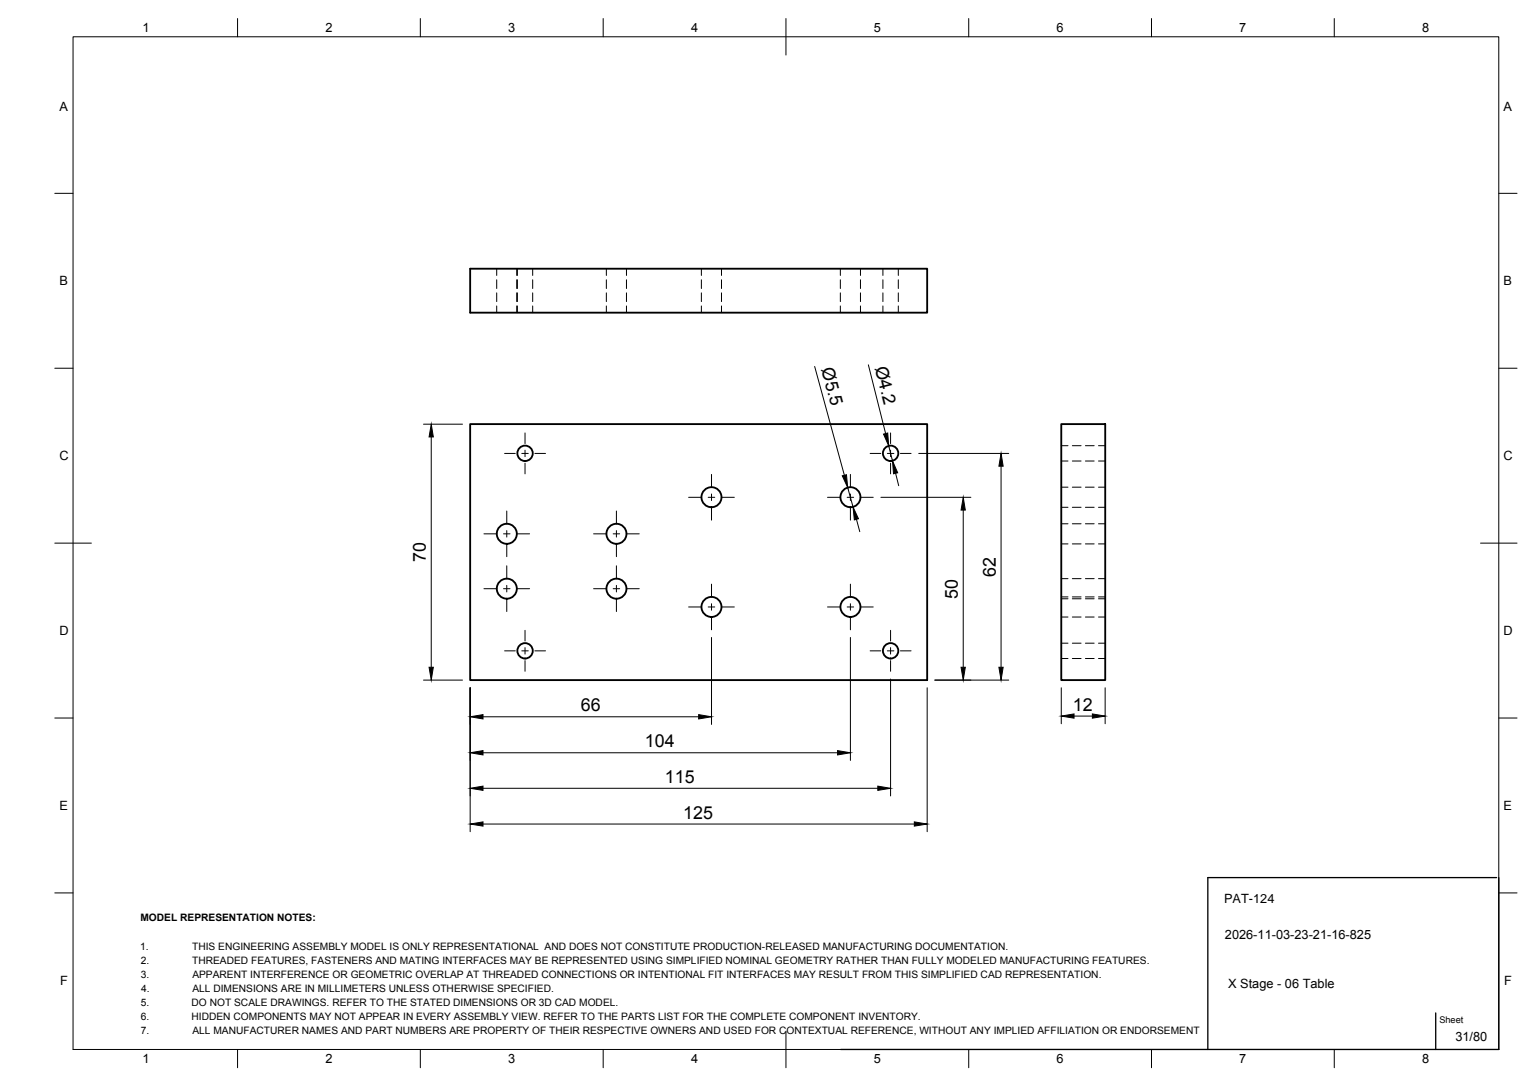
ISO-10303-21;
HEADER;
/* Generated by software containing ST-Developer
 * from STEP Tools, Inc. (www.steptools.com) 
 */

FILE_DESCRIPTION(
/* description */ ('XY cross-slide table'),
/* implementation_level */ '2;1');

FILE_NAME(
/* name */ 'X Stage - 06 Table.step',
/* time_stamp */ '2026-10-28T03:22:46-07:00',
/* author */ (''),
/* organization */ (''),
/* preprocessor_version */ 'ST-DEVELOPER v20.2',
/* originating_system */ 'Autodesk Translation Framework v15.17.0.0',
/* authorisation */ '');

FILE_SCHEMA (('AUTOMOTIVE_DESIGN { 1 0 10303 214 3 1 1 }'));
ENDSEC;

DATA;
#10=MECHANICAL_DESIGN_GEOMETRIC_PRESENTATION_REPRESENTATION('',(#1707),#62984);
#1526=SHAPE_REPRESENTATION_RELATIONSHIP('SRR','None',#63377,#1609);
#1609=ADVANCED_BREP_SHAPE_REPRESENTATION('',(#1820),#62914);
#1707=STYLED_ITEM('',(#63898),#1820);
#1820=MANIFOLD_SOLID_BREP('Body1',#23001);
#2009=FACE_BOUND('',#4578,.T.);
#2010=FACE_BOUND('',#4579,.T.);
#2011=FACE_BOUND('',#4580,.T.);
#2012=FACE_BOUND('',#4581,.T.);
#2013=FACE_BOUND('',#4582,.T.);
#2014=FACE_BOUND('',#4583,.T.);
#2015=FACE_BOUND('',#4584,.T.);
#2016=FACE_BOUND('',#4585,.T.);
#2017=FACE_BOUND('',#4586,.T.);
#2018=FACE_BOUND('',#4587,.T.);
#2019=FACE_BOUND('',#4588,.T.);
#2020=FACE_BOUND('',#4589,.T.);
#2021=FACE_BOUND('',#4591,.T.);
#2022=FACE_BOUND('',#4592,.T.);
#2023=FACE_BOUND('',#4593,.T.);
#2024=FACE_BOUND('',#4594,.T.);
#2025=FACE_BOUND('',#4595,.T.);
#2026=FACE_BOUND('',#4596,.T.);
#2027=FACE_BOUND('',#4597,.T.);
#2028=FACE_BOUND('',#4598,.T.);
#2029=FACE_BOUND('',#4599,.T.);
#2030=FACE_BOUND('',#4600,.T.);
#2031=FACE_BOUND('',#4601,.T.);
#2032=FACE_BOUND('',#4602,.T.);
#2420=PLANE('',#24604);
#2421=PLANE('',#24605);
#2422=PLANE('',#24606);
#2423=PLANE('',#24607);
#2424=PLANE('',#24608);
#2425=PLANE('',#24609);
#3125=FACE_OUTER_BOUND('',#4561,.T.);
#3126=FACE_OUTER_BOUND('',#4562,.T.);
#3127=FACE_OUTER_BOUND('',#4563,.T.);
#3128=FACE_OUTER_BOUND('',#4564,.T.);
#3129=FACE_OUTER_BOUND('',#4565,.T.);
#3130=FACE_OUTER_BOUND('',#4566,.T.);
#3131=FACE_OUTER_BOUND('',#4567,.T.);
#3132=FACE_OUTER_BOUND('',#4568,.T.);
#3133=FACE_OUTER_BOUND('',#4569,.T.);
#3134=FACE_OUTER_BOUND('',#4570,.T.);
#3135=FACE_OUTER_BOUND('',#4571,.T.);
#3136=FACE_OUTER_BOUND('',#4572,.T.);
#3137=FACE_OUTER_BOUND('',#4573,.T.);
#3138=FACE_OUTER_BOUND('',#4574,.T.);
#3139=FACE_OUTER_BOUND('',#4575,.T.);
#3140=FACE_OUTER_BOUND('',#4576,.T.);
#3141=FACE_OUTER_BOUND('',#4577,.T.);
#3142=FACE_OUTER_BOUND('',#4590,.T.);
#4561=EDGE_LOOP('',(#16012,#16013,#16014,#16015));
#4562=EDGE_LOOP('',(#16016,#16017,#16018,#16019));
#4563=EDGE_LOOP('',(#16020,#16021,#16022,#16023));
#4564=EDGE_LOOP('',(#16024,#16025,#16026,#16027));
#4565=EDGE_LOOP('',(#16028,#16029,#16030,#16031));
#4566=EDGE_LOOP('',(#16032,#16033,#16034,#16035));
#4567=EDGE_LOOP('',(#16036,#16037,#16038,#16039));
#4568=EDGE_LOOP('',(#16040,#16041,#16042,#16043));
#4569=EDGE_LOOP('',(#16044,#16045,#16046,#16047));
#4570=EDGE_LOOP('',(#16048,#16049,#16050,#16051));
#4571=EDGE_LOOP('',(#16052,#16053,#16054,#16055));
#4572=EDGE_LOOP('',(#16056,#16057,#16058,#16059));
#4573=EDGE_LOOP('',(#16060,#16061,#16062,#16063));
#4574=EDGE_LOOP('',(#16064,#16065,#16066,#16067));
#4575=EDGE_LOOP('',(#16068,#16069,#16070,#16071));
#4576=EDGE_LOOP('',(#16072,#16073,#16074,#16075));
#4577=EDGE_LOOP('',(#16076,#16077,#16078,#16079));
#4578=EDGE_LOOP('',(#16080));
#4579=EDGE_LOOP('',(#16081));
#4580=EDGE_LOOP('',(#16082));
#4581=EDGE_LOOP('',(#16083));
#4582=EDGE_LOOP('',(#16084));
#4583=EDGE_LOOP('',(#16085));
#4584=EDGE_LOOP('',(#16086));
#4585=EDGE_LOOP('',(#16087));
#4586=EDGE_LOOP('',(#16088));
#4587=EDGE_LOOP('',(#16089));
#4588=EDGE_LOOP('',(#16090));
#4589=EDGE_LOOP('',(#16091));
#4590=EDGE_LOOP('',(#16092,#16093,#16094,#16095));
#4591=EDGE_LOOP('',(#16096));
#4592=EDGE_LOOP('',(#16097));
#4593=EDGE_LOOP('',(#16098));
#4594=EDGE_LOOP('',(#16099));
#4595=EDGE_LOOP('',(#16100));
#4596=EDGE_LOOP('',(#16101));
#4597=EDGE_LOOP('',(#16102));
#4598=EDGE_LOOP('',(#16103));
#4599=EDGE_LOOP('',(#16104));
#4600=EDGE_LOOP('',(#16105));
#4601=EDGE_LOOP('',(#16106));
#4602=EDGE_LOOP('',(#16107));
#6155=LINE('',#34739,#7642);
#6156=LINE('',#34745,#7643);
#6157=LINE('',#34751,#7644);
#6158=LINE('',#34757,#7645);
#6159=LINE('',#34763,#7646);
#6160=LINE('',#34769,#7647);
#6161=LINE('',#34775,#7648);
#6162=LINE('',#34781,#7649);
#6163=LINE('',#34787,#7650);
#6164=LINE('',#34793,#7651);
#6165=LINE('',#34799,#7652);
#6166=LINE('',#34805,#7653);
#6167=LINE('',#34810,#7654);
#6168=LINE('',#34812,#7655);
#6169=LINE('',#34814,#7656);
#6170=LINE('',#34815,#7657);
#6171=LINE('',#34818,#7658);
#6172=LINE('',#34820,#7659);
#6173=LINE('',#34821,#7660);
#6174=LINE('',#34824,#7661);
#6175=LINE('',#34826,#7662);
#6176=LINE('',#34827,#7663);
#6177=LINE('',#34829,#7664);
#6178=LINE('',#34830,#7665);
#7642=VECTOR('',#27850,0.210000000000001);
#7643=VECTOR('',#27857,0.210000000000001);
#7644=VECTOR('',#27864,0.210000000000001);
#7645=VECTOR('',#27871,0.210000000000001);
#7646=VECTOR('',#27878,0.275);
#7647=VECTOR('',#27885,0.275);
#7648=VECTOR('',#27892,0.275);
#7649=VECTOR('',#27899,0.275);
#7650=VECTOR('',#27906,0.275);
#7651=VECTOR('',#27913,0.275);
#7652=VECTOR('',#27920,0.275);
#7653=VECTOR('',#27927,0.275);
#7654=VECTOR('',#27932,1.);
#7655=VECTOR('',#27933,1.);
#7656=VECTOR('',#27934,1.);
#7657=VECTOR('',#27935,1.);
#7658=VECTOR('',#27938,1.);
#7659=VECTOR('',#27939,1.);
#7660=VECTOR('',#27940,1.);
#7661=VECTOR('',#27943,1.);
#7662=VECTOR('',#27944,1.);
#7663=VECTOR('',#27945,1.);
#7664=VECTOR('',#27948,1.);
#7665=VECTOR('',#27949,1.);
#9153=CIRCLE('',#24569,0.210000000000001);
#9154=CIRCLE('',#24570,0.210000000000001);
#9155=CIRCLE('',#24572,0.210000000000001);
#9156=CIRCLE('',#24573,0.210000000000001);
#9157=CIRCLE('',#24575,0.210000000000001);
#9158=CIRCLE('',#24576,0.210000000000001);
#9159=CIRCLE('',#24578,0.210000000000001);
#9160=CIRCLE('',#24579,0.210000000000001);
#9161=CIRCLE('',#24581,0.275);
#9162=CIRCLE('',#24582,0.275);
#9163=CIRCLE('',#24584,0.275);
#9164=CIRCLE('',#24585,0.275);
#9165=CIRCLE('',#24587,0.275);
#9166=CIRCLE('',#24588,0.275);
#9167=CIRCLE('',#24590,0.275);
#9168=CIRCLE('',#24591,0.275);
#9169=CIRCLE('',#24593,0.275);
#9170=CIRCLE('',#24594,0.275);
#9171=CIRCLE('',#24596,0.275);
#9172=CIRCLE('',#24597,0.275);
#9173=CIRCLE('',#24599,0.275);
#9174=CIRCLE('',#24600,0.275);
#9175=CIRCLE('',#24602,0.275);
#9176=CIRCLE('',#24603,0.275);
#10157=VERTEX_POINT('',#34736);
#10158=VERTEX_POINT('',#34738);
#10159=VERTEX_POINT('',#34742);
#10160=VERTEX_POINT('',#34744);
#10161=VERTEX_POINT('',#34748);
#10162=VERTEX_POINT('',#34750);
#10163=VERTEX_POINT('',#34754);
#10164=VERTEX_POINT('',#34756);
#10165=VERTEX_POINT('',#34760);
#10166=VERTEX_POINT('',#34762);
#10167=VERTEX_POINT('',#34766);
#10168=VERTEX_POINT('',#34768);
#10169=VERTEX_POINT('',#34772);
#10170=VERTEX_POINT('',#34774);
#10171=VERTEX_POINT('',#34778);
#10172=VERTEX_POINT('',#34780);
#10173=VERTEX_POINT('',#34784);
#10174=VERTEX_POINT('',#34786);
#10175=VERTEX_POINT('',#34790);
#10176=VERTEX_POINT('',#34792);
#10177=VERTEX_POINT('',#34796);
#10178=VERTEX_POINT('',#34798);
#10179=VERTEX_POINT('',#34802);
#10180=VERTEX_POINT('',#34804);
#10181=VERTEX_POINT('',#34808);
#10182=VERTEX_POINT('',#34809);
#10183=VERTEX_POINT('',#34811);
#10184=VERTEX_POINT('',#34813);
#10185=VERTEX_POINT('',#34817);
#10186=VERTEX_POINT('',#34819);
#10187=VERTEX_POINT('',#34823);
#10188=VERTEX_POINT('',#34825);
#12390=EDGE_CURVE('',#10157,#10157,#9153,.T.);
#12391=EDGE_CURVE('',#10157,#10158,#6155,.T.);
#12392=EDGE_CURVE('',#10158,#10158,#9154,.T.);
#12393=EDGE_CURVE('',#10159,#10159,#9155,.T.);
#12394=EDGE_CURVE('',#10159,#10160,#6156,.T.);
#12395=EDGE_CURVE('',#10160,#10160,#9156,.T.);
#12396=EDGE_CURVE('',#10161,#10161,#9157,.T.);
#12397=EDGE_CURVE('',#10161,#10162,#6157,.T.);
#12398=EDGE_CURVE('',#10162,#10162,#9158,.T.);
#12399=EDGE_CURVE('',#10163,#10163,#9159,.T.);
#12400=EDGE_CURVE('',#10163,#10164,#6158,.T.);
#12401=EDGE_CURVE('',#10164,#10164,#9160,.T.);
#12402=EDGE_CURVE('',#10165,#10165,#9161,.T.);
#12403=EDGE_CURVE('',#10165,#10166,#6159,.T.);
#12404=EDGE_CURVE('',#10166,#10166,#9162,.T.);
#12405=EDGE_CURVE('',#10167,#10167,#9163,.T.);
#12406=EDGE_CURVE('',#10167,#10168,#6160,.T.);
#12407=EDGE_CURVE('',#10168,#10168,#9164,.T.);
#12408=EDGE_CURVE('',#10169,#10169,#9165,.T.);
#12409=EDGE_CURVE('',#10169,#10170,#6161,.T.);
#12410=EDGE_CURVE('',#10170,#10170,#9166,.T.);
#12411=EDGE_CURVE('',#10171,#10171,#9167,.T.);
#12412=EDGE_CURVE('',#10171,#10172,#6162,.T.);
#12413=EDGE_CURVE('',#10172,#10172,#9168,.T.);
#12414=EDGE_CURVE('',#10173,#10173,#9169,.T.);
#12415=EDGE_CURVE('',#10173,#10174,#6163,.T.);
#12416=EDGE_CURVE('',#10174,#10174,#9170,.T.);
#12417=EDGE_CURVE('',#10175,#10175,#9171,.T.);
#12418=EDGE_CURVE('',#10175,#10176,#6164,.T.);
#12419=EDGE_CURVE('',#10176,#10176,#9172,.T.);
#12420=EDGE_CURVE('',#10177,#10177,#9173,.T.);
#12421=EDGE_CURVE('',#10177,#10178,#6165,.T.);
#12422=EDGE_CURVE('',#10178,#10178,#9174,.T.);
#12423=EDGE_CURVE('',#10179,#10179,#9175,.T.);
#12424=EDGE_CURVE('',#10179,#10180,#6166,.T.);
#12425=EDGE_CURVE('',#10180,#10180,#9176,.T.);
#12426=EDGE_CURVE('',#10181,#10182,#6167,.T.);
#12427=EDGE_CURVE('',#10182,#10183,#6168,.T.);
#12428=EDGE_CURVE('',#10184,#10183,#6169,.T.);
#12429=EDGE_CURVE('',#10181,#10184,#6170,.T.);
#12430=EDGE_CURVE('',#10185,#10181,#6171,.T.);
#12431=EDGE_CURVE('',#10186,#10184,#6172,.T.);
#12432=EDGE_CURVE('',#10185,#10186,#6173,.T.);
#12433=EDGE_CURVE('',#10187,#10185,#6174,.T.);
#12434=EDGE_CURVE('',#10188,#10186,#6175,.T.);
#12435=EDGE_CURVE('',#10187,#10188,#6176,.T.);
#12436=EDGE_CURVE('',#10182,#10187,#6177,.T.);
#12437=EDGE_CURVE('',#10183,#10188,#6178,.T.);
#16012=ORIENTED_EDGE('',*,*,#12390,.F.);
#16013=ORIENTED_EDGE('',*,*,#12391,.T.);
#16014=ORIENTED_EDGE('',*,*,#12392,.F.);
#16015=ORIENTED_EDGE('',*,*,#12391,.F.);
#16016=ORIENTED_EDGE('',*,*,#12393,.F.);
#16017=ORIENTED_EDGE('',*,*,#12394,.T.);
#16018=ORIENTED_EDGE('',*,*,#12395,.F.);
#16019=ORIENTED_EDGE('',*,*,#12394,.F.);
#16020=ORIENTED_EDGE('',*,*,#12396,.F.);
#16021=ORIENTED_EDGE('',*,*,#12397,.T.);
#16022=ORIENTED_EDGE('',*,*,#12398,.F.);
#16023=ORIENTED_EDGE('',*,*,#12397,.F.);
#16024=ORIENTED_EDGE('',*,*,#12399,.F.);
#16025=ORIENTED_EDGE('',*,*,#12400,.T.);
#16026=ORIENTED_EDGE('',*,*,#12401,.F.);
#16027=ORIENTED_EDGE('',*,*,#12400,.F.);
#16028=ORIENTED_EDGE('',*,*,#12402,.F.);
#16029=ORIENTED_EDGE('',*,*,#12403,.T.);
#16030=ORIENTED_EDGE('',*,*,#12404,.F.);
#16031=ORIENTED_EDGE('',*,*,#12403,.F.);
#16032=ORIENTED_EDGE('',*,*,#12405,.F.);
#16033=ORIENTED_EDGE('',*,*,#12406,.T.);
#16034=ORIENTED_EDGE('',*,*,#12407,.F.);
#16035=ORIENTED_EDGE('',*,*,#12406,.F.);
#16036=ORIENTED_EDGE('',*,*,#12408,.F.);
#16037=ORIENTED_EDGE('',*,*,#12409,.T.);
#16038=ORIENTED_EDGE('',*,*,#12410,.F.);
#16039=ORIENTED_EDGE('',*,*,#12409,.F.);
#16040=ORIENTED_EDGE('',*,*,#12411,.F.);
#16041=ORIENTED_EDGE('',*,*,#12412,.T.);
#16042=ORIENTED_EDGE('',*,*,#12413,.F.);
#16043=ORIENTED_EDGE('',*,*,#12412,.F.);
#16044=ORIENTED_EDGE('',*,*,#12414,.F.);
#16045=ORIENTED_EDGE('',*,*,#12415,.T.);
#16046=ORIENTED_EDGE('',*,*,#12416,.F.);
#16047=ORIENTED_EDGE('',*,*,#12415,.F.);
#16048=ORIENTED_EDGE('',*,*,#12417,.F.);
#16049=ORIENTED_EDGE('',*,*,#12418,.T.);
#16050=ORIENTED_EDGE('',*,*,#12419,.F.);
#16051=ORIENTED_EDGE('',*,*,#12418,.F.);
#16052=ORIENTED_EDGE('',*,*,#12420,.F.);
#16053=ORIENTED_EDGE('',*,*,#12421,.T.);
#16054=ORIENTED_EDGE('',*,*,#12422,.F.);
#16055=ORIENTED_EDGE('',*,*,#12421,.F.);
#16056=ORIENTED_EDGE('',*,*,#12423,.F.);
#16057=ORIENTED_EDGE('',*,*,#12424,.T.);
#16058=ORIENTED_EDGE('',*,*,#12425,.F.);
#16059=ORIENTED_EDGE('',*,*,#12424,.F.);
#16060=ORIENTED_EDGE('',*,*,#12426,.T.);
#16061=ORIENTED_EDGE('',*,*,#12427,.T.);
#16062=ORIENTED_EDGE('',*,*,#12428,.F.);
#16063=ORIENTED_EDGE('',*,*,#12429,.F.);
#16064=ORIENTED_EDGE('',*,*,#12430,.T.);
#16065=ORIENTED_EDGE('',*,*,#12429,.T.);
#16066=ORIENTED_EDGE('',*,*,#12431,.F.);
#16067=ORIENTED_EDGE('',*,*,#12432,.F.);
#16068=ORIENTED_EDGE('',*,*,#12433,.T.);
#16069=ORIENTED_EDGE('',*,*,#12432,.T.);
#16070=ORIENTED_EDGE('',*,*,#12434,.F.);
#16071=ORIENTED_EDGE('',*,*,#12435,.F.);
#16072=ORIENTED_EDGE('',*,*,#12436,.T.);
#16073=ORIENTED_EDGE('',*,*,#12435,.T.);
#16074=ORIENTED_EDGE('',*,*,#12437,.F.);
#16075=ORIENTED_EDGE('',*,*,#12427,.F.);
#16076=ORIENTED_EDGE('',*,*,#12437,.T.);
#16077=ORIENTED_EDGE('',*,*,#12434,.T.);
#16078=ORIENTED_EDGE('',*,*,#12431,.T.);
#16079=ORIENTED_EDGE('',*,*,#12428,.T.);
#16080=ORIENTED_EDGE('',*,*,#12404,.T.);
#16081=ORIENTED_EDGE('',*,*,#12407,.T.);
#16082=ORIENTED_EDGE('',*,*,#12410,.T.);
#16083=ORIENTED_EDGE('',*,*,#12413,.T.);
#16084=ORIENTED_EDGE('',*,*,#12416,.T.);
#16085=ORIENTED_EDGE('',*,*,#12419,.T.);
#16086=ORIENTED_EDGE('',*,*,#12422,.T.);
#16087=ORIENTED_EDGE('',*,*,#12425,.T.);
#16088=ORIENTED_EDGE('',*,*,#12401,.T.);
#16089=ORIENTED_EDGE('',*,*,#12398,.T.);
#16090=ORIENTED_EDGE('',*,*,#12395,.T.);
#16091=ORIENTED_EDGE('',*,*,#12392,.T.);
#16092=ORIENTED_EDGE('',*,*,#12436,.F.);
#16093=ORIENTED_EDGE('',*,*,#12426,.F.);
#16094=ORIENTED_EDGE('',*,*,#12430,.F.);
#16095=ORIENTED_EDGE('',*,*,#12433,.F.);
#16096=ORIENTED_EDGE('',*,*,#12402,.T.);
#16097=ORIENTED_EDGE('',*,*,#12405,.T.);
#16098=ORIENTED_EDGE('',*,*,#12408,.T.);
#16099=ORIENTED_EDGE('',*,*,#12411,.T.);
#16100=ORIENTED_EDGE('',*,*,#12414,.T.);
#16101=ORIENTED_EDGE('',*,*,#12417,.T.);
#16102=ORIENTED_EDGE('',*,*,#12420,.T.);
#16103=ORIENTED_EDGE('',*,*,#12423,.T.);
#16104=ORIENTED_EDGE('',*,*,#12399,.T.);
#16105=ORIENTED_EDGE('',*,*,#12396,.T.);
#16106=ORIENTED_EDGE('',*,*,#12393,.T.);
#16107=ORIENTED_EDGE('',*,*,#12390,.T.);
#21130=CYLINDRICAL_SURFACE('',#24568,0.210000000000001);
#21131=CYLINDRICAL_SURFACE('',#24571,0.210000000000001);
#21132=CYLINDRICAL_SURFACE('',#24574,0.210000000000001);
#21133=CYLINDRICAL_SURFACE('',#24577,0.210000000000001);
#21134=CYLINDRICAL_SURFACE('',#24580,0.275);
#21135=CYLINDRICAL_SURFACE('',#24583,0.275);
#21136=CYLINDRICAL_SURFACE('',#24586,0.275);
#21137=CYLINDRICAL_SURFACE('',#24589,0.275);
#21138=CYLINDRICAL_SURFACE('',#24592,0.275);
#21139=CYLINDRICAL_SURFACE('',#24595,0.275);
#21140=CYLINDRICAL_SURFACE('',#24598,0.275);
#21141=CYLINDRICAL_SURFACE('',#24601,0.275);
#21906=ADVANCED_FACE('',(#3125),#21130,.F.);
#21907=ADVANCED_FACE('',(#3126),#21131,.F.);
#21908=ADVANCED_FACE('',(#3127),#21132,.F.);
#21909=ADVANCED_FACE('',(#3128),#21133,.F.);
#21910=ADVANCED_FACE('',(#3129),#21134,.F.);
#21911=ADVANCED_FACE('',(#3130),#21135,.F.);
#21912=ADVANCED_FACE('',(#3131),#21136,.F.);
#21913=ADVANCED_FACE('',(#3132),#21137,.F.);
#21914=ADVANCED_FACE('',(#3133),#21138,.F.);
#21915=ADVANCED_FACE('',(#3134),#21139,.F.);
#21916=ADVANCED_FACE('',(#3135),#21140,.F.);
#21917=ADVANCED_FACE('',(#3136),#21141,.F.);
#21918=ADVANCED_FACE('',(#3137),#2420,.T.);
#21919=ADVANCED_FACE('',(#3138),#2421,.T.);
#21920=ADVANCED_FACE('',(#3139),#2422,.T.);
#21921=ADVANCED_FACE('',(#3140),#2423,.T.);
#21922=ADVANCED_FACE('',(#3141,#2009,#2010,#2011,#2012,#2013,#2014,#2015,
#2016,#2017,#2018,#2019,#2020),#2424,.T.);
#21923=ADVANCED_FACE('',(#3142,#2021,#2022,#2023,#2024,#2025,#2026,#2027,
#2028,#2029,#2030,#2031,#2032),#2425,.F.);
#23001=CLOSED_SHELL('',(#21906,#21907,#21908,#21909,#21910,#21911,#21912,
#21913,#21914,#21915,#21916,#21917,#21918,#21919,#21920,#21921,#21922,#21923));
#24567=AXIS2_PLACEMENT_3D('',#34734,#27844,#27845);
#24568=AXIS2_PLACEMENT_3D('',#34735,#27846,#27847);
#24569=AXIS2_PLACEMENT_3D('',#34737,#27848,#27849);
#24570=AXIS2_PLACEMENT_3D('',#34740,#27851,#27852);
#24571=AXIS2_PLACEMENT_3D('',#34741,#27853,#27854);
#24572=AXIS2_PLACEMENT_3D('',#34743,#27855,#27856);
#24573=AXIS2_PLACEMENT_3D('',#34746,#27858,#27859);
#24574=AXIS2_PLACEMENT_3D('',#34747,#27860,#27861);
#24575=AXIS2_PLACEMENT_3D('',#34749,#27862,#27863);
#24576=AXIS2_PLACEMENT_3D('',#34752,#27865,#27866);
#24577=AXIS2_PLACEMENT_3D('',#34753,#27867,#27868);
#24578=AXIS2_PLACEMENT_3D('',#34755,#27869,#27870);
#24579=AXIS2_PLACEMENT_3D('',#34758,#27872,#27873);
#24580=AXIS2_PLACEMENT_3D('',#34759,#27874,#27875);
#24581=AXIS2_PLACEMENT_3D('',#34761,#27876,#27877);
#24582=AXIS2_PLACEMENT_3D('',#34764,#27879,#27880);
#24583=AXIS2_PLACEMENT_3D('',#34765,#27881,#27882);
#24584=AXIS2_PLACEMENT_3D('',#34767,#27883,#27884);
#24585=AXIS2_PLACEMENT_3D('',#34770,#27886,#27887);
#24586=AXIS2_PLACEMENT_3D('',#34771,#27888,#27889);
#24587=AXIS2_PLACEMENT_3D('',#34773,#27890,#27891);
#24588=AXIS2_PLACEMENT_3D('',#34776,#27893,#27894);
#24589=AXIS2_PLACEMENT_3D('',#34777,#27895,#27896);
#24590=AXIS2_PLACEMENT_3D('',#34779,#27897,#27898);
#24591=AXIS2_PLACEMENT_3D('',#34782,#27900,#27901);
#24592=AXIS2_PLACEMENT_3D('',#34783,#27902,#27903);
#24593=AXIS2_PLACEMENT_3D('',#34785,#27904,#27905);
#24594=AXIS2_PLACEMENT_3D('',#34788,#27907,#27908);
#24595=AXIS2_PLACEMENT_3D('',#34789,#27909,#27910);
#24596=AXIS2_PLACEMENT_3D('',#34791,#27911,#27912);
#24597=AXIS2_PLACEMENT_3D('',#34794,#27914,#27915);
#24598=AXIS2_PLACEMENT_3D('',#34795,#27916,#27917);
#24599=AXIS2_PLACEMENT_3D('',#34797,#27918,#27919);
#24600=AXIS2_PLACEMENT_3D('',#34800,#27921,#27922);
#24601=AXIS2_PLACEMENT_3D('',#34801,#27923,#27924);
#24602=AXIS2_PLACEMENT_3D('',#34803,#27925,#27926);
#24603=AXIS2_PLACEMENT_3D('',#34806,#27928,#27929);
#24604=AXIS2_PLACEMENT_3D('',#34807,#27930,#27931);
#24605=AXIS2_PLACEMENT_3D('',#34816,#27936,#27937);
#24606=AXIS2_PLACEMENT_3D('',#34822,#27941,#27942);
#24607=AXIS2_PLACEMENT_3D('',#34828,#27946,#27947);
#24608=AXIS2_PLACEMENT_3D('',#34831,#27950,#27951);
#24609=AXIS2_PLACEMENT_3D('',#34832,#27952,#27953);
#27844=DIRECTION('axis',(0.,0.,1.));
#27845=DIRECTION('refdir',(1.,0.,0.));
#27846=DIRECTION('center_axis',(0.,0.,1.));
#27847=DIRECTION('ref_axis',(1.,0.,0.));
#27848=DIRECTION('center_axis',(0.,0.,1.));
#27849=DIRECTION('ref_axis',(1.,0.,0.));
#27850=DIRECTION('',(0.,0.,1.));
#27851=DIRECTION('center_axis',(0.,0.,-1.));
#27852=DIRECTION('ref_axis',(1.,0.,0.));
#27853=DIRECTION('center_axis',(0.,0.,1.));
#27854=DIRECTION('ref_axis',(1.,0.,0.));
#27855=DIRECTION('center_axis',(0.,0.,1.));
#27856=DIRECTION('ref_axis',(1.,0.,0.));
#27857=DIRECTION('',(0.,0.,1.));
#27858=DIRECTION('center_axis',(0.,0.,-1.));
#27859=DIRECTION('ref_axis',(1.,0.,0.));
#27860=DIRECTION('center_axis',(0.,0.,1.));
#27861=DIRECTION('ref_axis',(1.,0.,0.));
#27862=DIRECTION('center_axis',(0.,0.,1.));
#27863=DIRECTION('ref_axis',(1.,0.,0.));
#27864=DIRECTION('',(0.,0.,1.));
#27865=DIRECTION('center_axis',(0.,0.,-1.));
#27866=DIRECTION('ref_axis',(1.,0.,0.));
#27867=DIRECTION('center_axis',(0.,0.,1.));
#27868=DIRECTION('ref_axis',(1.,0.,0.));
#27869=DIRECTION('center_axis',(0.,0.,1.));
#27870=DIRECTION('ref_axis',(1.,0.,0.));
#27871=DIRECTION('',(0.,0.,1.));
#27872=DIRECTION('center_axis',(0.,0.,-1.));
#27873=DIRECTION('ref_axis',(1.,0.,0.));
#27874=DIRECTION('center_axis',(0.,0.,1.));
#27875=DIRECTION('ref_axis',(1.,0.,0.));
#27876=DIRECTION('center_axis',(0.,0.,1.));
#27877=DIRECTION('ref_axis',(1.,0.,0.));
#27878=DIRECTION('',(0.,0.,1.));
#27879=DIRECTION('center_axis',(0.,0.,-1.));
#27880=DIRECTION('ref_axis',(1.,0.,0.));
#27881=DIRECTION('center_axis',(0.,0.,1.));
#27882=DIRECTION('ref_axis',(1.,0.,0.));
#27883=DIRECTION('center_axis',(0.,0.,1.));
#27884=DIRECTION('ref_axis',(1.,0.,0.));
#27885=DIRECTION('',(0.,0.,1.));
#27886=DIRECTION('center_axis',(0.,0.,-1.));
#27887=DIRECTION('ref_axis',(1.,0.,0.));
#27888=DIRECTION('center_axis',(0.,0.,1.));
#27889=DIRECTION('ref_axis',(1.,0.,0.));
#27890=DIRECTION('center_axis',(0.,0.,1.));
#27891=DIRECTION('ref_axis',(1.,0.,0.));
#27892=DIRECTION('',(0.,0.,1.));
#27893=DIRECTION('center_axis',(0.,0.,-1.));
#27894=DIRECTION('ref_axis',(1.,0.,0.));
#27895=DIRECTION('center_axis',(0.,0.,1.));
#27896=DIRECTION('ref_axis',(1.,0.,0.));
#27897=DIRECTION('center_axis',(0.,0.,1.));
#27898=DIRECTION('ref_axis',(1.,0.,0.));
#27899=DIRECTION('',(0.,0.,1.));
#27900=DIRECTION('center_axis',(0.,0.,-1.));
#27901=DIRECTION('ref_axis',(1.,0.,0.));
#27902=DIRECTION('center_axis',(0.,0.,1.));
#27903=DIRECTION('ref_axis',(1.,0.,0.));
#27904=DIRECTION('center_axis',(0.,0.,1.));
#27905=DIRECTION('ref_axis',(1.,0.,0.));
#27906=DIRECTION('',(0.,0.,1.));
#27907=DIRECTION('center_axis',(0.,0.,-1.));
#27908=DIRECTION('ref_axis',(1.,0.,0.));
#27909=DIRECTION('center_axis',(0.,0.,1.));
#27910=DIRECTION('ref_axis',(1.,0.,0.));
#27911=DIRECTION('center_axis',(0.,0.,1.));
#27912=DIRECTION('ref_axis',(1.,0.,0.));
#27913=DIRECTION('',(0.,0.,1.));
#27914=DIRECTION('center_axis',(0.,0.,-1.));
#27915=DIRECTION('ref_axis',(1.,0.,0.));
#27916=DIRECTION('center_axis',(0.,0.,1.));
#27917=DIRECTION('ref_axis',(1.,0.,0.));
#27918=DIRECTION('center_axis',(0.,0.,1.));
#27919=DIRECTION('ref_axis',(1.,0.,0.));
#27920=DIRECTION('',(0.,0.,1.));
#27921=DIRECTION('center_axis',(0.,0.,-1.));
#27922=DIRECTION('ref_axis',(1.,0.,0.));
#27923=DIRECTION('center_axis',(0.,0.,1.));
#27924=DIRECTION('ref_axis',(1.,0.,0.));
#27925=DIRECTION('center_axis',(0.,0.,1.));
#27926=DIRECTION('ref_axis',(1.,0.,0.));
#27927=DIRECTION('',(0.,0.,1.));
#27928=DIRECTION('center_axis',(0.,0.,-1.));
#27929=DIRECTION('ref_axis',(1.,0.,0.));
#27930=DIRECTION('center_axis',(0.,1.,0.));
#27931=DIRECTION('ref_axis',(-1.,0.,0.));
#27932=DIRECTION('',(-1.,0.,0.));
#27933=DIRECTION('',(0.,0.,1.));
#27934=DIRECTION('',(-1.,0.,0.));
#27935=DIRECTION('',(0.,0.,1.));
#27936=DIRECTION('center_axis',(1.,0.,0.));
#27937=DIRECTION('ref_axis',(0.,1.,0.));
#27938=DIRECTION('',(0.,1.,0.));
#27939=DIRECTION('',(0.,1.,0.));
#27940=DIRECTION('',(0.,0.,1.));
#27941=DIRECTION('center_axis',(0.,-1.,0.));
#27942=DIRECTION('ref_axis',(1.,0.,0.));
#27943=DIRECTION('',(1.,0.,0.));
#27944=DIRECTION('',(1.,0.,0.));
#27945=DIRECTION('',(0.,0.,1.));
#27946=DIRECTION('center_axis',(-1.,0.,0.));
#27947=DIRECTION('ref_axis',(0.,-1.,0.));
#27948=DIRECTION('',(0.,-1.,0.));
#27949=DIRECTION('',(0.,-1.,0.));
#27950=DIRECTION('center_axis',(0.,0.,1.));
#27951=DIRECTION('ref_axis',(1.,0.,0.));
#27952=DIRECTION('center_axis',(0.,0.,1.));
#27953=DIRECTION('ref_axis',(1.,0.,0.));
#34734=CARTESIAN_POINT('',(0.,0.,0.));
#34735=CARTESIAN_POINT('Origin',(16.2,-9.,5.9));
#34736=CARTESIAN_POINT('',(15.99,-9.,6.));
#34737=CARTESIAN_POINT('Origin',(16.2,-9.,6.));
#34738=CARTESIAN_POINT('',(15.99,-9.,7.2));
#34739=CARTESIAN_POINT('',(15.99,-9.,5.9));
#34740=CARTESIAN_POINT('Origin',(16.2,-9.,7.2));
#34741=CARTESIAN_POINT('Origin',(10.8,1.,5.9));
#34742=CARTESIAN_POINT('',(10.59,1.,6.));
#34743=CARTESIAN_POINT('Origin',(10.8,1.,6.));
#34744=CARTESIAN_POINT('',(10.59,1.,7.2));
#34745=CARTESIAN_POINT('',(10.59,1.,5.9));
#34746=CARTESIAN_POINT('Origin',(10.8,1.,7.2));
#34747=CARTESIAN_POINT('Origin',(10.8,-9.,5.9));
#34748=CARTESIAN_POINT('',(10.59,-9.,6.));
#34749=CARTESIAN_POINT('Origin',(10.8,-9.,6.));
#34750=CARTESIAN_POINT('',(10.59,-9.,7.2));
#34751=CARTESIAN_POINT('',(10.59,-9.,5.9));
#34752=CARTESIAN_POINT('Origin',(10.8,-9.,7.2));
#34753=CARTESIAN_POINT('Origin',(16.2,1.,5.9));
#34754=CARTESIAN_POINT('',(15.99,1.,6.));
#34755=CARTESIAN_POINT('Origin',(16.2,1.,6.));
#34756=CARTESIAN_POINT('',(15.99,1.,7.2));
#34757=CARTESIAN_POINT('',(15.99,1.,5.9));
#34758=CARTESIAN_POINT('Origin',(16.2,1.,7.2));
#34759=CARTESIAN_POINT('Origin',(14.,-1.5,5.9));
#34760=CARTESIAN_POINT('',(13.725,-1.5,6.));
#34761=CARTESIAN_POINT('Origin',(14.,-1.5,6.));
#34762=CARTESIAN_POINT('',(13.725,-1.5,7.2));
#34763=CARTESIAN_POINT('',(13.725,-1.5,5.9));
#34764=CARTESIAN_POINT('Origin',(14.,-1.5,7.2));
#34765=CARTESIAN_POINT('Origin',(12.5,1.5,5.9));
#34766=CARTESIAN_POINT('',(12.225,1.5,6.));
#34767=CARTESIAN_POINT('Origin',(12.5,1.5,6.));
#34768=CARTESIAN_POINT('',(12.225,1.5,7.2));
#34769=CARTESIAN_POINT('',(12.225,1.5,5.9));
#34770=CARTESIAN_POINT('Origin',(12.5,1.5,7.2));
#34771=CARTESIAN_POINT('Origin',(12.5,-1.5,5.9));
#34772=CARTESIAN_POINT('',(12.225,-1.5,6.));
#34773=CARTESIAN_POINT('Origin',(12.5,-1.5,6.));
#34774=CARTESIAN_POINT('',(12.225,-1.5,7.2));
#34775=CARTESIAN_POINT('',(12.225,-1.5,5.9));
#34776=CARTESIAN_POINT('Origin',(12.5,-1.5,7.2));
#34777=CARTESIAN_POINT('Origin',(14.,1.5,5.9));
#34778=CARTESIAN_POINT('',(13.725,1.5,6.));
#34779=CARTESIAN_POINT('Origin',(14.,1.5,6.));
#34780=CARTESIAN_POINT('',(13.725,1.5,7.2));
#34781=CARTESIAN_POINT('',(13.725,1.5,5.9));
#34782=CARTESIAN_POINT('Origin',(14.,1.5,7.2));
#34783=CARTESIAN_POINT('Origin',(15.,-7.9,5.1));
#34784=CARTESIAN_POINT('',(14.725,-7.9,6.));
#34785=CARTESIAN_POINT('Origin',(15.,-7.9,6.));
#34786=CARTESIAN_POINT('',(14.725,-7.9,7.2));
#34787=CARTESIAN_POINT('',(14.725,-7.9,5.1));
#34788=CARTESIAN_POINT('Origin',(15.,-7.9,7.2));
#34789=CARTESIAN_POINT('Origin',(12.,-4.1,5.1));
#34790=CARTESIAN_POINT('',(11.725,-4.1,6.));
#34791=CARTESIAN_POINT('Origin',(12.,-4.1,6.));
#34792=CARTESIAN_POINT('',(11.725,-4.1,7.2));
#34793=CARTESIAN_POINT('',(11.725,-4.1,5.1));
#34794=CARTESIAN_POINT('Origin',(12.,-4.1,7.2));
#34795=CARTESIAN_POINT('Origin',(12.,-7.9,5.1));
#34796=CARTESIAN_POINT('',(11.725,-7.9,6.));
#34797=CARTESIAN_POINT('Origin',(12.,-7.9,6.));
#34798=CARTESIAN_POINT('',(11.725,-7.9,7.2));
#34799=CARTESIAN_POINT('',(11.725,-7.9,5.1));
#34800=CARTESIAN_POINT('Origin',(12.,-7.9,7.2));
#34801=CARTESIAN_POINT('Origin',(15.,-4.1,5.1));
#34802=CARTESIAN_POINT('',(14.725,-4.1,6.));
#34803=CARTESIAN_POINT('Origin',(15.,-4.1,6.));
#34804=CARTESIAN_POINT('',(14.725,-4.1,7.2));
#34805=CARTESIAN_POINT('',(14.725,-4.1,5.1));
#34806=CARTESIAN_POINT('Origin',(15.,-4.1,7.2));
#34807=CARTESIAN_POINT('Origin',(17.,2.5,6.));
#34808=CARTESIAN_POINT('',(17.,2.5,6.));
#34809=CARTESIAN_POINT('',(10.,2.5,6.));
#34810=CARTESIAN_POINT('',(17.,2.5,6.));
#34811=CARTESIAN_POINT('',(10.,2.5,7.2));
#34812=CARTESIAN_POINT('',(10.,2.5,6.));
#34813=CARTESIAN_POINT('',(17.,2.5,7.2));
#34814=CARTESIAN_POINT('',(17.,2.5,7.2));
#34815=CARTESIAN_POINT('',(17.,2.5,6.));
#34816=CARTESIAN_POINT('Origin',(17.,-10.,6.));
#34817=CARTESIAN_POINT('',(17.,-10.,6.));
#34818=CARTESIAN_POINT('',(17.,-10.,6.));
#34819=CARTESIAN_POINT('',(17.,-10.,7.2));
#34820=CARTESIAN_POINT('',(17.,-10.,7.2));
#34821=CARTESIAN_POINT('',(17.,-10.,6.));
#34822=CARTESIAN_POINT('Origin',(10.,-10.,6.));
#34823=CARTESIAN_POINT('',(10.,-10.,6.));
#34824=CARTESIAN_POINT('',(10.,-10.,6.));
#34825=CARTESIAN_POINT('',(10.,-10.,7.2));
#34826=CARTESIAN_POINT('',(10.,-10.,7.2));
#34827=CARTESIAN_POINT('',(10.,-10.,6.));
#34828=CARTESIAN_POINT('Origin',(10.,2.5,6.));
#34829=CARTESIAN_POINT('',(10.,2.5,6.));
#34830=CARTESIAN_POINT('',(10.,2.5,7.2));
#34831=CARTESIAN_POINT('Origin',(13.5,-3.75,7.2));
#34832=CARTESIAN_POINT('Origin',(13.5,-3.75,6.));
#62815=UNCERTAINTY_MEASURE_WITH_UNIT(LENGTH_MEASURE(0.001),#62985,
'DISTANCE_ACCURACY_VALUE',
'Maximum model space distance between geometric entities at asserted c
onnectivities');
#62885=UNCERTAINTY_MEASURE_WITH_UNIT(LENGTH_MEASURE(0.001),#62985,
'DISTANCE_ACCURACY_VALUE',
'Maximum model space distance between geometric entities at asserted c
onnectivities');
#62914=(
GEOMETRIC_REPRESENTATION_CONTEXT(3)
GLOBAL_UNCERTAINTY_ASSIGNED_CONTEXT((#62815))
GLOBAL_UNIT_ASSIGNED_CONTEXT((#62985,#62987,#62988))
REPRESENTATION_CONTEXT('','3D')
);
#62984=(
GEOMETRIC_REPRESENTATION_CONTEXT(3)
GLOBAL_UNCERTAINTY_ASSIGNED_CONTEXT((#62885))
GLOBAL_UNIT_ASSIGNED_CONTEXT((#62985,#62987,#62988))
REPRESENTATION_CONTEXT('','3D')
);
#62985=(
LENGTH_UNIT()
NAMED_UNIT(*)
SI_UNIT(.CENTI.,.METRE.)
);
#62987=(
NAMED_UNIT(*)
PLANE_ANGLE_UNIT()
SI_UNIT($,.RADIAN.)
);
#62988=(
NAMED_UNIT(*)
SI_UNIT($,.STERADIAN.)
SOLID_ANGLE_UNIT()
);
#63017=SHAPE_DEFINITION_REPRESENTATION(#63125,#63377);
#63125=PRODUCT_DEFINITION_SHAPE('',$,#63476);
#63377=SHAPE_REPRESENTATION('',(#24567),#62914);
#63447=PRODUCT_DEFINITION_CONTEXT('part definition',#63743,'design');
#63476=PRODUCT_DEFINITION('X Stage - 06 Table','X Stage - 06 Table',#63574,
#63447);
#63574=PRODUCT_DEFINITION_FORMATION('',$,#63773);
#63743=APPLICATION_CONTEXT(
'Core Data for Automotive Mechanical Design Process');
#63744=PRODUCT_CONTEXT('part definition',#63743,'mechanical');
#63773=PRODUCT('X Stage - 06 Table','X Stage - 06 Table',
'X Stage - 06 Table',(#63744));
#63892=COLOUR_RGB('Light Blue',0.38,0.62,0.78);
#63893=FILL_AREA_STYLE_COLOUR('',#63892);
#63894=FILL_AREA_STYLE('',(#63893));
#63895=SURFACE_STYLE_FILL_AREA(#63894);
#63896=SURFACE_SIDE_STYLE('',(#63895));
#63897=SURFACE_STYLE_USAGE(.BOTH.,#63896);
#63898=PRESENTATION_STYLE_ASSIGNMENT((#63897));
ENDSEC;
END-ISO-10303-21;
